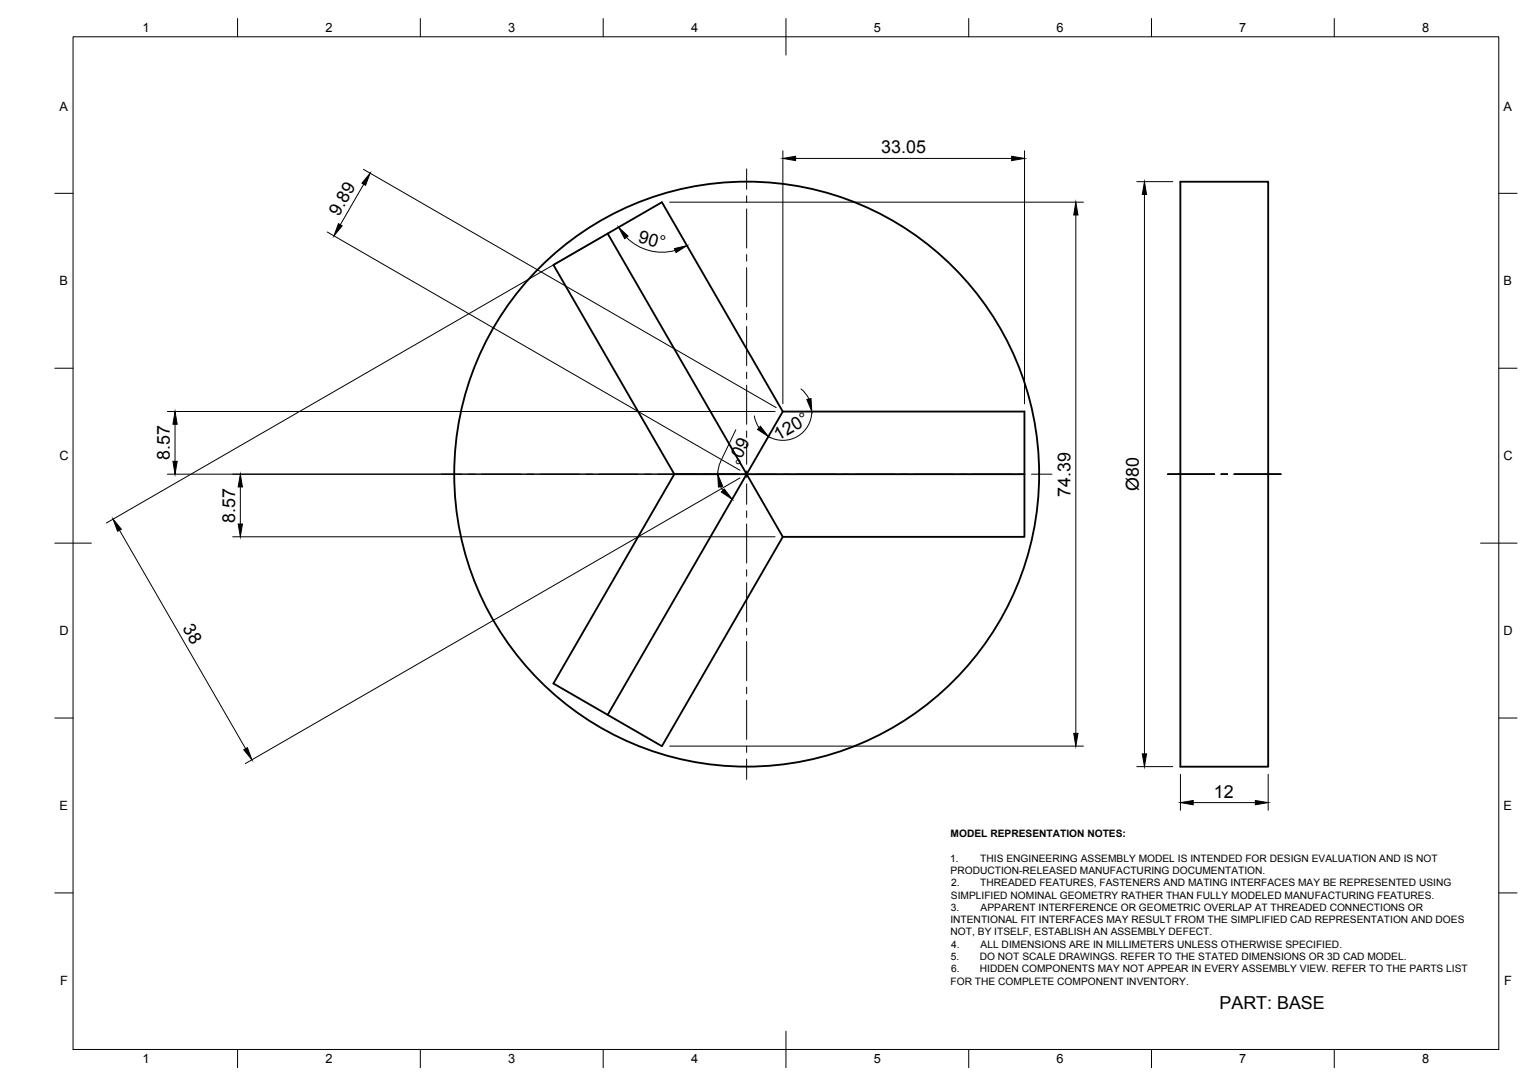
ISO-10303-21;
HEADER;
/* Generated by software containing ST-Developer
 * from STEP Tools, Inc. (www.steptools.com) 
 */

FILE_DESCRIPTION(
/* description */ (''),
/* implementation_level */ '2;1');

FILE_NAME(
/* name */ 'Base.step',
/* time_stamp */ '2026-10-05T00:14:20-07:00',
/* author */ (''),
/* organization */ (''),
/* preprocessor_version */ 'ST-DEVELOPER v20.2',
/* originating_system */ 'Autodesk Translation Framework v15.15.0.0',
/* authorisation */ '');

FILE_SCHEMA (('AUTOMOTIVE_DESIGN { 1 0 10303 214 3 1 1 }'));
ENDSEC;

DATA;
#10=MECHANICAL_DESIGN_GEOMETRIC_PRESENTATION_REPRESENTATION('',(#3371),#75336);
#3355=SHAPE_REPRESENTATION_RELATIONSHIP('SRR','None',#75368,#3363);
#3363=ADVANCED_BREP_SHAPE_REPRESENTATION('',(#3379),#75328);
#3371=STYLED_ITEM('',(#75417),#3379);
#3379=MANIFOLD_SOLID_BREP('Body1',#32021);
#3387=FACE_BOUND('',#6872,.T.);
#3400=CIRCLE('',#32130,40.);
#3401=CIRCLE('',#32131,40.);
#4455=CYLINDRICAL_SURFACE('',#32129,40.);
#5134=FACE_OUTER_BOUND('',#6861,.T.);
#5135=FACE_OUTER_BOUND('',#6862,.T.);
#5136=FACE_OUTER_BOUND('',#6863,.T.);
#5137=FACE_OUTER_BOUND('',#6864,.T.);
#5138=FACE_OUTER_BOUND('',#6865,.T.);
#5139=FACE_OUTER_BOUND('',#6866,.T.);
#5140=FACE_OUTER_BOUND('',#6867,.T.);
#5141=FACE_OUTER_BOUND('',#6868,.T.);
#5142=FACE_OUTER_BOUND('',#6869,.T.);
#5143=FACE_OUTER_BOUND('',#6870,.T.);
#5144=FACE_OUTER_BOUND('',#6871,.T.);
#5145=FACE_OUTER_BOUND('',#6873,.T.);
#6861=EDGE_LOOP('',(#19577,#19578,#19579,#19580));
#6862=EDGE_LOOP('',(#19581,#19582,#19583,#19584));
#6863=EDGE_LOOP('',(#19585,#19586,#19587,#19588));
#6864=EDGE_LOOP('',(#19589,#19590,#19591));
#6865=EDGE_LOOP('',(#19592,#19593,#19594,#19595));
#6866=EDGE_LOOP('',(#19596,#19597,#19598));
#6867=EDGE_LOOP('',(#19599,#19600,#19601,#19602));
#6868=EDGE_LOOP('',(#19603,#19604,#19605,#19606));
#6869=EDGE_LOOP('',(#19607,#19608,#19609));
#6870=EDGE_LOOP('',(#19610,#19611,#19612,#19613));
#6871=EDGE_LOOP('',(#19614));
#6872=EDGE_LOOP('',(#19615,#19616,#19617,#19618,#19619,#19620,#19621,#19622,
#19623));
#6873=EDGE_LOOP('',(#19624));
#8601=LINE('',#46050,#9847);
#8602=LINE('',#46052,#9848);
#8603=LINE('',#46054,#9849);
#8604=LINE('',#46055,#9850);
#8605=LINE('',#46058,#9851);
#8606=LINE('',#46060,#9852);
#8607=LINE('',#46062,#9853);
#8608=LINE('',#46063,#9854);
#8609=LINE('',#46066,#9855);
#8610=LINE('',#46068,#9856);
#8611=LINE('',#46069,#9857);
#8612=LINE('',#46071,#9858);
#8613=LINE('',#46074,#9859);
#8614=LINE('',#46075,#9860);
#8615=LINE('',#46077,#9861);
#8616=LINE('',#46080,#9862);
#8617=LINE('',#46082,#9863);
#8618=LINE('',#46083,#9864);
#8619=LINE('',#46086,#9865);
#8620=LINE('',#46087,#9866);
#8621=LINE('',#46089,#9867);
#8622=LINE('',#46094,#9868);
#9847=VECTOR('',#36351,10.);
#9848=VECTOR('',#36352,10.);
#9849=VECTOR('',#36353,10.);
#9850=VECTOR('',#36354,10.);
#9851=VECTOR('',#36357,10.);
#9852=VECTOR('',#36358,9.99999999999999);
#9853=VECTOR('',#36359,10.);
#9854=VECTOR('',#36360,9.99999999999999);
#9855=VECTOR('',#36363,10.);
#9856=VECTOR('',#36364,10.);
#9857=VECTOR('',#36365,9.99999999999999);
#9858=VECTOR('',#36368,10.);
#9859=VECTOR('',#36371,10.);
#9860=VECTOR('',#36372,10.);
#9861=VECTOR('',#36375,10.);
#9862=VECTOR('',#36378,10.);
#9863=VECTOR('',#36379,10.);
#9864=VECTOR('',#36380,10.);
#9865=VECTOR('',#36383,10.);
#9866=VECTOR('',#36384,10.);
#9867=VECTOR('',#36387,10.);
#9868=VECTOR('',#36392,40.);
#11093=VERTEX_POINT('',#46048);
#11094=VERTEX_POINT('',#46049);
#11095=VERTEX_POINT('',#46051);
#11096=VERTEX_POINT('',#46053);
#11097=VERTEX_POINT('',#46057);
#11098=VERTEX_POINT('',#46059);
#11099=VERTEX_POINT('',#46061);
#11100=VERTEX_POINT('',#46065);
#11101=VERTEX_POINT('',#46067);
#11102=VERTEX_POINT('',#46073);
#11103=VERTEX_POINT('',#46079);
#11104=VERTEX_POINT('',#46081);
#11105=VERTEX_POINT('',#46085);
#11106=VERTEX_POINT('',#46091);
#11107=VERTEX_POINT('',#46093);
#14483=EDGE_CURVE('',#11093,#11094,#8601,.T.);
#14484=EDGE_CURVE('',#11095,#11093,#8602,.T.);
#14485=EDGE_CURVE('',#11095,#11096,#8603,.T.);
#14486=EDGE_CURVE('',#11094,#11096,#8604,.T.);
#14487=EDGE_CURVE('',#11094,#11097,#8605,.T.);
#14488=EDGE_CURVE('',#11098,#11097,#8606,.T.);
#14489=EDGE_CURVE('',#11098,#11099,#8607,.T.);
#14490=EDGE_CURVE('',#11094,#11099,#8608,.T.);
#14491=EDGE_CURVE('',#11094,#11100,#8609,.T.);
#14492=EDGE_CURVE('',#11099,#11101,#8610,.T.);
#14493=EDGE_CURVE('',#11100,#11101,#8611,.T.);
#14494=EDGE_CURVE('',#11101,#11098,#8612,.T.);
#14495=EDGE_CURVE('',#11096,#11102,#8613,.T.);
#14496=EDGE_CURVE('',#11097,#11102,#8614,.T.);
#14497=EDGE_CURVE('',#11102,#11095,#8615,.T.);
#14498=EDGE_CURVE('',#11094,#11103,#8616,.T.);
#14499=EDGE_CURVE('',#11103,#11104,#8617,.T.);
#14500=EDGE_CURVE('',#11093,#11104,#8618,.T.);
#14501=EDGE_CURVE('',#11105,#11100,#8619,.T.);
#14502=EDGE_CURVE('',#11105,#11103,#8620,.T.);
#14503=EDGE_CURVE('',#11104,#11105,#8621,.T.);
#14504=EDGE_CURVE('',#11106,#11106,#3400,.T.);
#14505=EDGE_CURVE('',#11106,#11107,#8622,.T.);
#14506=EDGE_CURVE('',#11107,#11107,#3401,.T.);
#19577=ORIENTED_EDGE('',*,*,#14483,.F.);
#19578=ORIENTED_EDGE('',*,*,#14484,.F.);
#19579=ORIENTED_EDGE('',*,*,#14485,.T.);
#19580=ORIENTED_EDGE('',*,*,#14486,.F.);
#19581=ORIENTED_EDGE('',*,*,#14487,.T.);
#19582=ORIENTED_EDGE('',*,*,#14488,.F.);
#19583=ORIENTED_EDGE('',*,*,#14489,.T.);
#19584=ORIENTED_EDGE('',*,*,#14490,.F.);
#19585=ORIENTED_EDGE('',*,*,#14491,.F.);
#19586=ORIENTED_EDGE('',*,*,#14490,.T.);
#19587=ORIENTED_EDGE('',*,*,#14492,.T.);
#19588=ORIENTED_EDGE('',*,*,#14493,.F.);
#19589=ORIENTED_EDGE('',*,*,#14492,.F.);
#19590=ORIENTED_EDGE('',*,*,#14489,.F.);
#19591=ORIENTED_EDGE('',*,*,#14494,.F.);
#19592=ORIENTED_EDGE('',*,*,#14487,.F.);
#19593=ORIENTED_EDGE('',*,*,#14486,.T.);
#19594=ORIENTED_EDGE('',*,*,#14495,.T.);
#19595=ORIENTED_EDGE('',*,*,#14496,.F.);
#19596=ORIENTED_EDGE('',*,*,#14495,.F.);
#19597=ORIENTED_EDGE('',*,*,#14485,.F.);
#19598=ORIENTED_EDGE('',*,*,#14497,.F.);
#19599=ORIENTED_EDGE('',*,*,#14483,.T.);
#19600=ORIENTED_EDGE('',*,*,#14498,.T.);
#19601=ORIENTED_EDGE('',*,*,#14499,.T.);
#19602=ORIENTED_EDGE('',*,*,#14500,.F.);
#19603=ORIENTED_EDGE('',*,*,#14491,.T.);
#19604=ORIENTED_EDGE('',*,*,#14501,.F.);
#19605=ORIENTED_EDGE('',*,*,#14502,.T.);
#19606=ORIENTED_EDGE('',*,*,#14498,.F.);
#19607=ORIENTED_EDGE('',*,*,#14499,.F.);
#19608=ORIENTED_EDGE('',*,*,#14502,.F.);
#19609=ORIENTED_EDGE('',*,*,#14503,.F.);
#19610=ORIENTED_EDGE('',*,*,#14504,.F.);
#19611=ORIENTED_EDGE('',*,*,#14505,.T.);
#19612=ORIENTED_EDGE('',*,*,#14506,.T.);
#19613=ORIENTED_EDGE('',*,*,#14505,.F.);
#19614=ORIENTED_EDGE('',*,*,#14504,.T.);
#19615=ORIENTED_EDGE('',*,*,#14484,.T.);
#19616=ORIENTED_EDGE('',*,*,#14500,.T.);
#19617=ORIENTED_EDGE('',*,*,#14503,.T.);
#19618=ORIENTED_EDGE('',*,*,#14501,.T.);
#19619=ORIENTED_EDGE('',*,*,#14493,.T.);
#19620=ORIENTED_EDGE('',*,*,#14494,.T.);
#19621=ORIENTED_EDGE('',*,*,#14488,.T.);
#19622=ORIENTED_EDGE('',*,*,#14496,.T.);
#19623=ORIENTED_EDGE('',*,*,#14497,.T.);
#19624=ORIENTED_EDGE('',*,*,#14506,.F.);
#29765=PLANE('',#32120);
#29766=PLANE('',#32121);
#29767=PLANE('',#32122);
#29768=PLANE('',#32123);
#29769=PLANE('',#32124);
#29770=PLANE('',#32125);
#29771=PLANE('',#32126);
#29772=PLANE('',#32127);
#29773=PLANE('',#32128);
#29774=PLANE('',#32132);
#29775=PLANE('',#32133);
#30294=ADVANCED_FACE('',(#5134),#29765,.F.);
#30295=ADVANCED_FACE('',(#5135),#29766,.F.);
#30296=ADVANCED_FACE('',(#5136),#29767,.F.);
#30297=ADVANCED_FACE('',(#5137),#29768,.F.);
#30298=ADVANCED_FACE('',(#5138),#29769,.F.);
#30299=ADVANCED_FACE('',(#5139),#29770,.F.);
#30300=ADVANCED_FACE('',(#5140),#29771,.F.);
#30301=ADVANCED_FACE('',(#5141),#29772,.F.);
#30302=ADVANCED_FACE('',(#5142),#29773,.F.);
#30303=ADVANCED_FACE('',(#5143),#4455,.T.);
#30304=ADVANCED_FACE('',(#5144,#3387),#29774,.T.);
#30305=ADVANCED_FACE('',(#5145),#29775,.F.);
#32021=CLOSED_SHELL('',(#30294,#30295,#30296,#30297,#30298,#30299,#30300,
#30301,#30302,#30303,#30304,#30305));
#32119=AXIS2_PLACEMENT_3D('',#46046,#36347,#36348);
#32120=AXIS2_PLACEMENT_3D('',#46047,#36349,#36350);
#32121=AXIS2_PLACEMENT_3D('',#46056,#36355,#36356);
#32122=AXIS2_PLACEMENT_3D('',#46064,#36361,#36362);
#32123=AXIS2_PLACEMENT_3D('',#46070,#36366,#36367);
#32124=AXIS2_PLACEMENT_3D('',#46072,#36369,#36370);
#32125=AXIS2_PLACEMENT_3D('',#46076,#36373,#36374);
#32126=AXIS2_PLACEMENT_3D('',#46078,#36376,#36377);
#32127=AXIS2_PLACEMENT_3D('',#46084,#36381,#36382);
#32128=AXIS2_PLACEMENT_3D('',#46088,#36385,#36386);
#32129=AXIS2_PLACEMENT_3D('',#46090,#36388,#36389);
#32130=AXIS2_PLACEMENT_3D('',#46092,#36390,#36391);
#32131=AXIS2_PLACEMENT_3D('',#46095,#36393,#36394);
#32132=AXIS2_PLACEMENT_3D('',#46096,#36395,#36396);
#32133=AXIS2_PLACEMENT_3D('',#46097,#36397,#36398);
#36347=DIRECTION('axis',(0.,0.,1.));
#36348=DIRECTION('refdir',(1.,0.,0.));
#36349=DIRECTION('center_axis',(0.496731764892154,0.286788218175523,-0.819152044288992));
#36350=DIRECTION('ref_axis',(-0.709406479916223,-0.409576022144496,-0.573576436351046));
#36351=DIRECTION('',(-0.427535056636437,-0.740512440111147,-0.51851239270389));
#36352=DIRECTION('',(0.5,-0.866025403784439,0.));
#36353=DIRECTION('',(-0.709406479916223,-0.409576022144496,-0.573576436351046));
#36354=DIRECTION('',(-0.5,0.866025403784439,0.));
#36355=DIRECTION('center_axis',(-0.496731764892154,0.286788218175523,-0.819152044288992));
#36356=DIRECTION('ref_axis',(0.709406479916223,-0.409576022144496,-0.573576436351046));
#36357=DIRECTION('',(-0.855070113272875,2.22044604925031E-16,0.51851239270389));
#36358=DIRECTION('',(0.5,0.866025403784439,0.));
#36359=DIRECTION('',(0.709406479916223,-0.409576022144496,-0.573576436351045));
#36360=DIRECTION('',(-0.5,-0.866025403784439,0.));
#36361=DIRECTION('center_axis',(0.496731764892154,-0.286788218175523,-0.819152044288992));
#36362=DIRECTION('ref_axis',(0.709406479916223,-0.409576022144496,0.573576436351046));
#36363=DIRECTION('',(0.427535056636437,-0.740512440111147,0.518512392703891));
#36364=DIRECTION('',(0.709406479916223,-0.409576022144496,0.573576436351045));
#36365=DIRECTION('',(-0.5,-0.866025403784439,0.));
#36366=DIRECTION('center_axis',(-0.500000000000001,-0.866025403784438,0.));
#36367=DIRECTION('ref_axis',(0.,0.,-1.));
#36368=DIRECTION('',(-0.866025403784438,0.5,0.));
#36369=DIRECTION('center_axis',(-0.496731764892154,-0.286788218175523,-0.819152044288992));
#36370=DIRECTION('ref_axis',(-0.709406479916223,-0.409576022144496,0.573576436351046));
#36371=DIRECTION('',(-0.709406479916223,-0.409576022144496,0.573576436351046));
#36372=DIRECTION('',(-0.5,0.866025403784439,0.));
#36373=DIRECTION('center_axis',(-0.5,0.866025403784439,0.));
#36374=DIRECTION('ref_axis',(0.,0.,-1.));
#36375=DIRECTION('',(0.866025403784439,0.5,0.));
#36376=DIRECTION('center_axis',(0.,0.573576436351046,-0.819152044288992));
#36377=DIRECTION('ref_axis',(0.,0.819152044288992,0.573576436351046));
#36378=DIRECTION('',(1.,0.,0.));
#36379=DIRECTION('',(0.,0.819152044288992,0.573576436351046));
#36380=DIRECTION('',(1.,0.,0.));
#36381=DIRECTION('center_axis',(0.,-0.573576436351046,-0.819152044288992));
#36382=DIRECTION('ref_axis',(0.,0.819152044288992,-0.573576436351046));
#36383=DIRECTION('',(-1.,0.,0.));
#36384=DIRECTION('',(0.,0.819152044288992,-0.573576436351046));
#36385=DIRECTION('center_axis',(1.,0.,0.));
#36386=DIRECTION('ref_axis',(0.,0.,-1.));
#36387=DIRECTION('',(0.,-1.,0.));
#36388=DIRECTION('center_axis',(0.,0.,1.));
#36389=DIRECTION('ref_axis',(1.,0.,0.));
#36390=DIRECTION('center_axis',(0.,0.,1.));
#36391=DIRECTION('ref_axis',(1.,0.,0.));
#36392=DIRECTION('',(0.,0.,-1.));
#36393=DIRECTION('center_axis',(0.,0.,1.));
#36394=DIRECTION('ref_axis',(1.,0.,0.));
#36395=DIRECTION('center_axis',(0.,0.,1.));
#36396=DIRECTION('ref_axis',(1.,0.,0.));
#36397=DIRECTION('center_axis',(0.,0.,1.));
#36398=DIRECTION('ref_axis',(1.,0.,0.));
#46046=CARTESIAN_POINT('',(0.,0.,0.));
#46047=CARTESIAN_POINT('Origin',(7.4208747252167,4.28444402022635,12.));
#46048=CARTESIAN_POINT('',(4.94724981681114,8.56888804045271,12.));
#46049=CARTESIAN_POINT('',(0.,0.,6.));
#46050=CARTESIAN_POINT('',(2.02148035019019,3.50130667303153,8.45164132604064));
#46051=CARTESIAN_POINT('',(-11.5791252747833,37.193409364035,12.));
#46052=CARTESIAN_POINT('',(7.4208747252167,4.28444402022635,12.));
#46053=CARTESIAN_POINT('',(-19.,32.9089653438087,6.));
#46054=CARTESIAN_POINT('',(-19.,32.9089653438087,6.));
#46055=CARTESIAN_POINT('',(0.,0.,6.));
#46056=CARTESIAN_POINT('Origin',(-7.4208747252167,4.28444402022636,12.));
#46057=CARTESIAN_POINT('',(-9.89449963362226,3.88578058618805E-15,12.));
#46058=CARTESIAN_POINT('',(-4.04296070038038,1.66533453693773E-15,8.45164132604064));
#46059=CARTESIAN_POINT('',(-26.4208747252167,-28.6245213235823,12.));
#46060=CARTESIAN_POINT('',(-7.4208747252167,4.28444402022635,12.));
#46061=CARTESIAN_POINT('',(-19.,-32.9089653438087,6.));
#46062=CARTESIAN_POINT('',(-19.,-32.9089653438087,6.));
#46063=CARTESIAN_POINT('',(0.,0.,6.));
#46064=CARTESIAN_POINT('Origin',(0.,0.,6.));
#46065=CARTESIAN_POINT('',(4.94724981681113,-8.5688880404527,12.));
#46066=CARTESIAN_POINT('',(2.02148035019019,-3.50130667303154,8.45164132604064));
#46067=CARTESIAN_POINT('',(-11.5791252747833,-37.193409364035,12.));
#46068=CARTESIAN_POINT('',(-19.,-32.9089653438087,6.));
#46069=CARTESIAN_POINT('',(7.4208747252167,-4.28444402022635,12.));
#46070=CARTESIAN_POINT('Origin',(-19.,-32.9089653438087,9.));
#46071=CARTESIAN_POINT('',(-19.,-32.9089653438087,12.));
#46072=CARTESIAN_POINT('Origin',(0.,0.,6.));
#46073=CARTESIAN_POINT('',(-26.4208747252167,28.6245213235823,12.));
#46074=CARTESIAN_POINT('',(-19.,32.9089653438087,6.));
#46075=CARTESIAN_POINT('',(-7.4208747252167,-4.28444402022635,12.));
#46076=CARTESIAN_POINT('Origin',(-19.,32.9089653438087,9.));
#46077=CARTESIAN_POINT('',(-19.,32.9089653438087,12.));
#46078=CARTESIAN_POINT('Origin',(0.,0.,6.));
#46079=CARTESIAN_POINT('',(38.,0.,6.));
#46080=CARTESIAN_POINT('',(0.,0.,6.));
#46081=CARTESIAN_POINT('',(38.,8.5688880404527,12.));
#46082=CARTESIAN_POINT('',(38.,0.,6.));
#46083=CARTESIAN_POINT('',(0.,8.5688880404527,12.));
#46084=CARTESIAN_POINT('Origin',(0.,-8.56888804045271,12.));
#46085=CARTESIAN_POINT('',(38.,-8.56888804045271,12.));
#46086=CARTESIAN_POINT('',(0.,-8.5688880404527,12.));
#46087=CARTESIAN_POINT('',(38.,0.,6.));
#46088=CARTESIAN_POINT('Origin',(38.,1.11022302462516E-15,9.));
#46089=CARTESIAN_POINT('',(38.,5.55111512312578E-16,12.));
#46090=CARTESIAN_POINT('Origin',(0.,0.,0.));
#46091=CARTESIAN_POINT('',(-40.,-4.89858719658941E-15,12.));
#46092=CARTESIAN_POINT('Origin',(0.,0.,12.));
#46093=CARTESIAN_POINT('',(-40.,-4.89858719658941E-15,0.));
#46094=CARTESIAN_POINT('',(-40.,-4.89858719658941E-15,0.));
#46095=CARTESIAN_POINT('Origin',(0.,0.,0.));
#46096=CARTESIAN_POINT('Origin',(0.,0.,12.));
#46097=CARTESIAN_POINT('Origin',(0.,0.,0.));
#75318=UNCERTAINTY_MEASURE_WITH_UNIT(LENGTH_MEASURE(0.01),#75337,
'DISTANCE_ACCURACY_VALUE',
'Maximum model space distance between geometric entities at asserted c
onnectivities');
#75326=UNCERTAINTY_MEASURE_WITH_UNIT(LENGTH_MEASURE(0.01),#75337,
'DISTANCE_ACCURACY_VALUE',
'Maximum model space distance between geometric entities at asserted c
onnectivities');
#75328=(
GEOMETRIC_REPRESENTATION_CONTEXT(3)
GLOBAL_UNCERTAINTY_ASSIGNED_CONTEXT((#75318))
GLOBAL_UNIT_ASSIGNED_CONTEXT((#75337,#75339,#75340))
REPRESENTATION_CONTEXT('','3D')
);
#75336=(
GEOMETRIC_REPRESENTATION_CONTEXT(3)
GLOBAL_UNCERTAINTY_ASSIGNED_CONTEXT((#75326))
GLOBAL_UNIT_ASSIGNED_CONTEXT((#75337,#75339,#75340))
REPRESENTATION_CONTEXT('','3D')
);
#75337=(
LENGTH_UNIT()
NAMED_UNIT(*)
SI_UNIT(.MILLI.,.METRE.)
);
#75339=(
NAMED_UNIT(*)
PLANE_ANGLE_UNIT()
SI_UNIT($,.RADIAN.)
);
#75340=(
NAMED_UNIT(*)
SI_UNIT($,.STERADIAN.)
SOLID_ANGLE_UNIT()
);
#75342=SHAPE_DEFINITION_REPRESENTATION(#75351,#75368);
#75351=PRODUCT_DEFINITION_SHAPE('',$,#75378);
#75368=SHAPE_REPRESENTATION('',(#32119),#75328);
#75376=PRODUCT_DEFINITION_CONTEXT('part definition',#75405,'design');
#75378=PRODUCT_DEFINITION('base','Base',#75387,#75376);
#75387=PRODUCT_DEFINITION_FORMATION('',$,#75408);
#75405=APPLICATION_CONTEXT(
'Core Data for Automotive Mechanical Design Process');
#75406=PRODUCT_CONTEXT('part definition',#75405,'mechanical');
#75408=PRODUCT('base','Base',$,(#75406));
#75417=PRESENTATION_STYLE_ASSIGNMENT((#75421));
#75421=SURFACE_STYLE_USAGE(.BOTH.,#75425);
#75425=SURFACE_SIDE_STYLE('',(#75429));
#75429=SURFACE_STYLE_FILL_AREA(#75433);
#75433=FILL_AREA_STYLE('Opaque(203,203,203)',(#75437));
#75437=FILL_AREA_STYLE_COLOUR('Opaque(203,203,203)',#75441);
#75441=COLOUR_RGB('Opaque(203,203,203)', 0.09019608, 0.27058824, 0.51372549);
ENDSEC;
END-ISO-10303-21;
